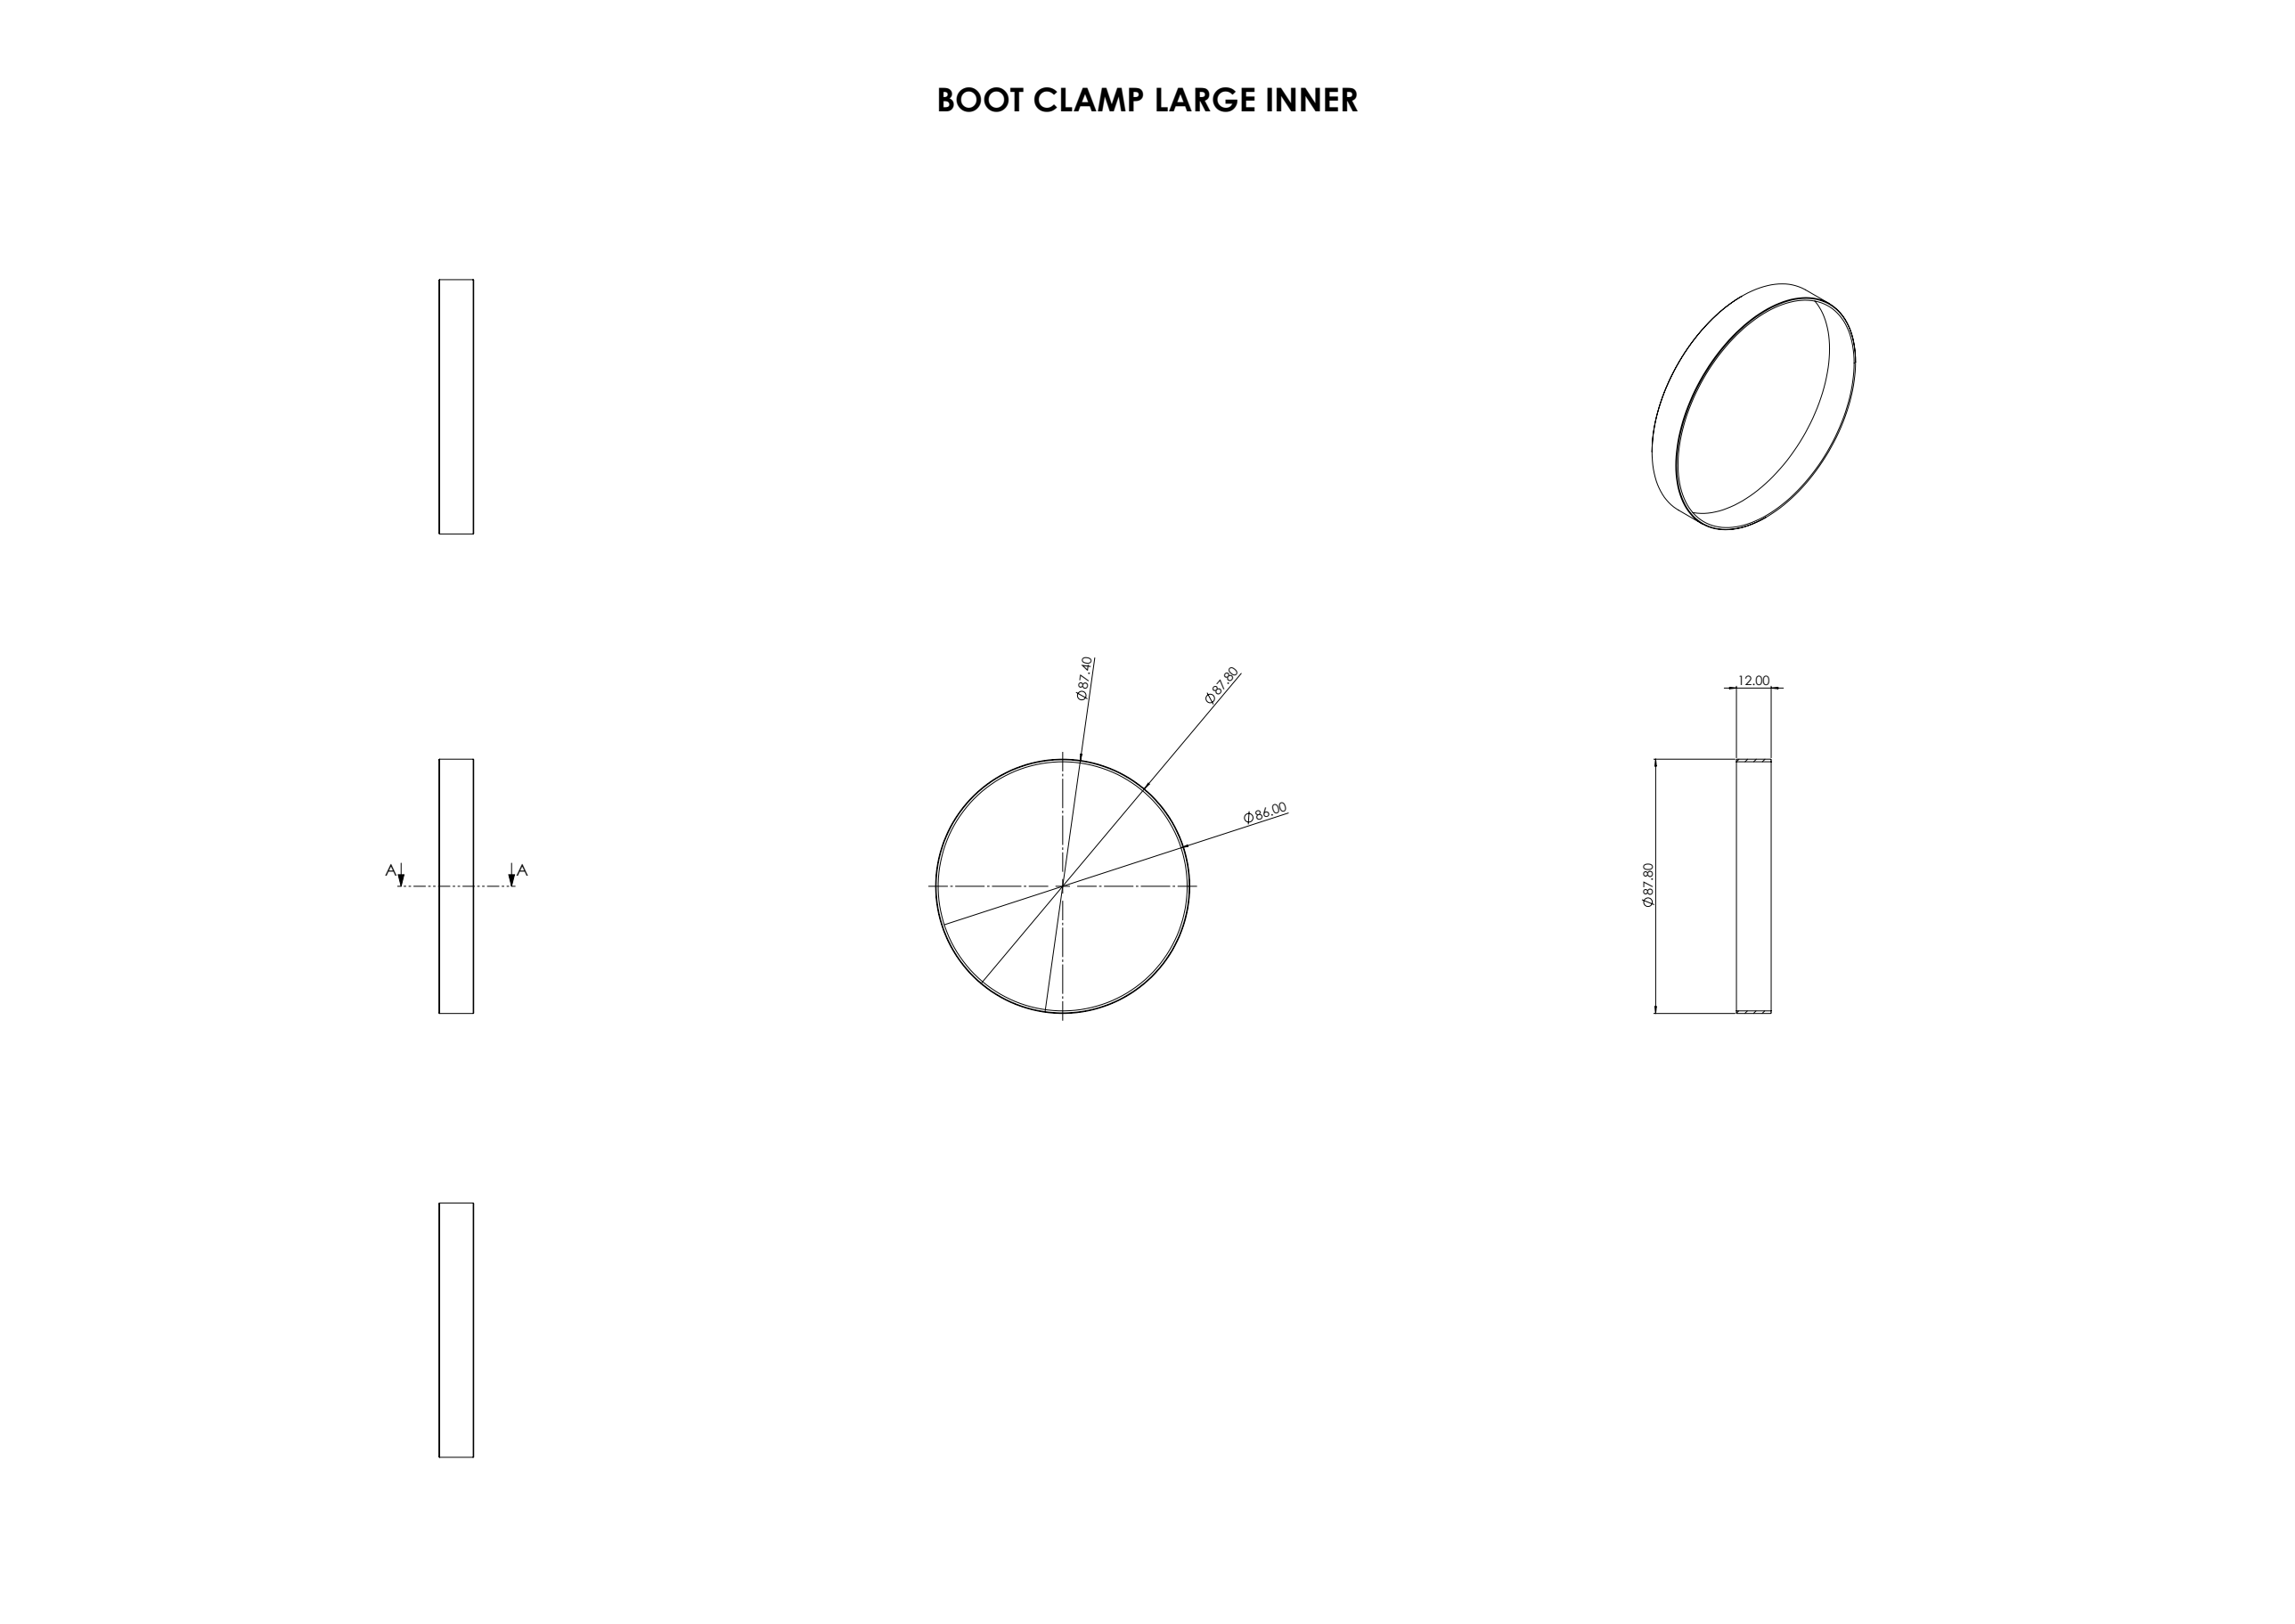
ISO-10303-21;
HEADER;
/* Generated by software containing ST-Developer
 * from STEP Tools, Inc. (www.steptools.com) 
 */

FILE_DESCRIPTION(
/* description */ (''),
/* implementation_level */ '2;1');

FILE_NAME(
/* name */ '12_Boot_Clamp_Large_Inner.step',
/* time_stamp */ '2026-10-11T12:57:03-07:00',
/* author */ (''),
/* organization */ (''),
/* preprocessor_version */ 'ST-DEVELOPER v20.2',
/* originating_system */ 'Autodesk Translation Framework v15.15.0.0',
/* authorisation */ '');

FILE_SCHEMA (('AUTOMOTIVE_DESIGN { 1 0 10303 214 3 1 1 }'));
ENDSEC;

DATA;
#10=MECHANICAL_DESIGN_GEOMETRIC_PRESENTATION_REPRESENTATION('',(#267),#90374);
#233=SHAPE_REPRESENTATION_RELATIONSHIP('SRR','None',#90452,#250);
#250=ADVANCED_BREP_SHAPE_REPRESENTATION('',(#284),#90368);
#267=STYLED_ITEM('',(#90673),#284);
#284=MANIFOLD_SOLID_BREP('Body1',#40356);
#743=CONICAL_SURFACE('',#44259,43.8,0.785398163397559);
#744=CONICAL_SURFACE('',#44264,43.8,0.785398163397382);
#1075=FACE_BOUND('',#6518,.T.);
#1076=FACE_BOUND('',#6521,.T.);
#1639=PLANE('',#44266);
#1640=PLANE('',#44270);
#4082=FACE_OUTER_BOUND('',#6514,.T.);
#4083=FACE_OUTER_BOUND('',#6515,.T.);
#4084=FACE_OUTER_BOUND('',#6516,.T.);
#4085=FACE_OUTER_BOUND('',#6517,.T.);
#4086=FACE_OUTER_BOUND('',#6519,.T.);
#4087=FACE_OUTER_BOUND('',#6520,.T.);
#6514=EDGE_LOOP('',(#34841,#34842,#34843,#34844));
#6515=EDGE_LOOP('',(#34845,#34846,#34847,#34848));
#6516=EDGE_LOOP('',(#34849,#34850,#34851,#34852));
#6517=EDGE_LOOP('',(#34853));
#6518=EDGE_LOOP('',(#34854));
#6519=EDGE_LOOP('',(#34855,#34856,#34857,#34858));
#6520=EDGE_LOOP('',(#34859));
#6521=EDGE_LOOP('',(#34860));
#8865=CIRCLE('',#44260,43.9);
#8866=CIRCLE('',#44261,43.7);
#8867=CIRCLE('',#44263,43.9);
#8868=CIRCLE('',#44265,43.7);
#8869=CIRCLE('',#44267,43.);
#8870=CIRCLE('',#44269,43.);
#12342=LINE('',#86910,#14836);
#12343=LINE('',#86915,#14837);
#12344=LINE('',#86919,#14838);
#12345=LINE('',#86925,#14839);
#14836=VECTOR('',#54702,43.8);
#14837=VECTOR('',#54709,43.9);
#14838=VECTOR('',#54714,43.8);
#14839=VECTOR('',#54721,43.);
#18296=VERTEX_POINT('',#86907);
#18297=VERTEX_POINT('',#86909);
#18298=VERTEX_POINT('',#86913);
#18299=VERTEX_POINT('',#86917);
#18300=VERTEX_POINT('',#86921);
#18301=VERTEX_POINT('',#86924);
#23932=EDGE_CURVE('',#18296,#18296,#8865,.T.);
#23933=EDGE_CURVE('',#18296,#18297,#12342,.T.);
#23934=EDGE_CURVE('',#18297,#18297,#8866,.T.);
#23935=EDGE_CURVE('',#18298,#18298,#8867,.T.);
#23936=EDGE_CURVE('',#18298,#18296,#12343,.T.);
#23937=EDGE_CURVE('',#18299,#18299,#8868,.T.);
#23938=EDGE_CURVE('',#18299,#18298,#12344,.T.);
#23939=EDGE_CURVE('',#18300,#18300,#8869,.T.);
#23940=EDGE_CURVE('',#18300,#18301,#12345,.T.);
#23941=EDGE_CURVE('',#18301,#18301,#8870,.T.);
#34841=ORIENTED_EDGE('',*,*,#23932,.F.);
#34842=ORIENTED_EDGE('',*,*,#23933,.T.);
#34843=ORIENTED_EDGE('',*,*,#23934,.T.);
#34844=ORIENTED_EDGE('',*,*,#23933,.F.);
#34845=ORIENTED_EDGE('',*,*,#23935,.F.);
#34846=ORIENTED_EDGE('',*,*,#23936,.T.);
#34847=ORIENTED_EDGE('',*,*,#23932,.T.);
#34848=ORIENTED_EDGE('',*,*,#23936,.F.);
#34849=ORIENTED_EDGE('',*,*,#23937,.F.);
#34850=ORIENTED_EDGE('',*,*,#23938,.T.);
#34851=ORIENTED_EDGE('',*,*,#23935,.T.);
#34852=ORIENTED_EDGE('',*,*,#23938,.F.);
#34853=ORIENTED_EDGE('',*,*,#23937,.T.);
#34854=ORIENTED_EDGE('',*,*,#23939,.F.);
#34855=ORIENTED_EDGE('',*,*,#23939,.T.);
#34856=ORIENTED_EDGE('',*,*,#23940,.T.);
#34857=ORIENTED_EDGE('',*,*,#23941,.F.);
#34858=ORIENTED_EDGE('',*,*,#23940,.F.);
#34859=ORIENTED_EDGE('',*,*,#23934,.F.);
#34860=ORIENTED_EDGE('',*,*,#23941,.T.);
#37783=CYLINDRICAL_SURFACE('',#44262,43.9);
#37784=CYLINDRICAL_SURFACE('',#44268,43.);
#39885=ADVANCED_FACE('',(#4082),#743,.T.);
#39886=ADVANCED_FACE('',(#4083),#37783,.T.);
#39887=ADVANCED_FACE('',(#4084),#744,.T.);
#39888=ADVANCED_FACE('',(#4085,#1075),#1639,.T.);
#39889=ADVANCED_FACE('',(#4086),#37784,.F.);
#39890=ADVANCED_FACE('',(#4087,#1076),#1640,.T.);
#40356=CLOSED_SHELL('',(#39885,#39886,#39887,#39888,#39889,#39890));
#44258=AXIS2_PLACEMENT_3D('',#86905,#54696,#54697);
#44259=AXIS2_PLACEMENT_3D('',#86906,#54698,#54699);
#44260=AXIS2_PLACEMENT_3D('',#86908,#54700,#54701);
#44261=AXIS2_PLACEMENT_3D('',#86911,#54703,#54704);
#44262=AXIS2_PLACEMENT_3D('',#86912,#54705,#54706);
#44263=AXIS2_PLACEMENT_3D('',#86914,#54707,#54708);
#44264=AXIS2_PLACEMENT_3D('',#86916,#54710,#54711);
#44265=AXIS2_PLACEMENT_3D('',#86918,#54712,#54713);
#44266=AXIS2_PLACEMENT_3D('',#86920,#54715,#54716);
#44267=AXIS2_PLACEMENT_3D('',#86922,#54717,#54718);
#44268=AXIS2_PLACEMENT_3D('',#86923,#54719,#54720);
#44269=AXIS2_PLACEMENT_3D('',#86926,#54722,#54723);
#44270=AXIS2_PLACEMENT_3D('',#86927,#54724,#54725);
#54696=DIRECTION('axis',(0.,0.,1.));
#54697=DIRECTION('refdir',(1.,0.,0.));
#54698=DIRECTION('center_axis',(1.,0.,0.));
#54699=DIRECTION('ref_axis',(0.,1.,0.));
#54700=DIRECTION('center_axis',(1.,0.,0.));
#54701=DIRECTION('ref_axis',(0.,0.,-1.));
#54702=DIRECTION('',(-0.707106781186469,0.707106781186626,8.65956056235589E-17));
#54703=DIRECTION('center_axis',(1.,0.,0.));
#54704=DIRECTION('ref_axis',(0.,0.,-1.));
#54705=DIRECTION('center_axis',(1.,0.,0.));
#54706=DIRECTION('ref_axis',(0.,1.,0.));
#54707=DIRECTION('center_axis',(1.,0.,0.));
#54708=DIRECTION('ref_axis',(0.,0.,-1.));
#54709=DIRECTION('',(-1.,0.,0.));
#54710=DIRECTION('center_axis',(-1.,0.,0.));
#54711=DIRECTION('ref_axis',(0.,1.,0.));
#54712=DIRECTION('center_axis',(1.,0.,0.));
#54713=DIRECTION('ref_axis',(0.,0.,-1.));
#54714=DIRECTION('',(-0.707106781186595,-0.7071067811865,-8.65956056235436E-17));
#54715=DIRECTION('center_axis',(1.,0.,0.));
#54716=DIRECTION('ref_axis',(0.,0.,-1.));
#54717=DIRECTION('center_axis',(1.,0.,0.));
#54718=DIRECTION('ref_axis',(0.,0.,-1.));
#54719=DIRECTION('center_axis',(1.,0.,0.));
#54720=DIRECTION('ref_axis',(0.,1.,0.));
#54721=DIRECTION('',(-1.,0.,0.));
#54722=DIRECTION('center_axis',(1.,0.,0.));
#54723=DIRECTION('ref_axis',(0.,0.,-1.));
#54724=DIRECTION('center_axis',(-1.,0.,0.));
#54725=DIRECTION('ref_axis',(0.,0.,1.));
#86905=CARTESIAN_POINT('',(0.,0.,0.));
#86906=CARTESIAN_POINT('Origin',(501.1,0.,0.));
#86907=CARTESIAN_POINT('',(501.2,-43.9,-5.37619944825688E-15));
#86908=CARTESIAN_POINT('Origin',(501.2,0.,0.));
#86909=CARTESIAN_POINT('',(501.,-43.7,-5.35170651227393E-15));
#86910=CARTESIAN_POINT('',(501.1,-43.8,-5.36395298026541E-15));
#86911=CARTESIAN_POINT('Origin',(501.,0.,0.));
#86912=CARTESIAN_POINT('Origin',(507.,0.,0.));
#86913=CARTESIAN_POINT('',(512.8,-43.9,-5.37619944825688E-15));
#86914=CARTESIAN_POINT('Origin',(512.8,0.,0.));
#86915=CARTESIAN_POINT('',(507.,-43.9,-5.37619944825688E-15));
#86916=CARTESIAN_POINT('Origin',(512.9,0.,0.));
#86917=CARTESIAN_POINT('',(513.,-43.7,-5.35170651227393E-15));
#86918=CARTESIAN_POINT('Origin',(513.,0.,0.));
#86919=CARTESIAN_POINT('',(512.9,-43.8,-5.36395298026541E-15));
#86920=CARTESIAN_POINT('Origin',(513.,43.,0.));
#86921=CARTESIAN_POINT('',(513.,-43.,-5.26598123633362E-15));
#86922=CARTESIAN_POINT('Origin',(513.,0.,0.));
#86923=CARTESIAN_POINT('Origin',(507.,0.,0.));
#86924=CARTESIAN_POINT('',(501.,-43.,-5.26598123633362E-15));
#86925=CARTESIAN_POINT('',(507.,-43.,-5.26598123633362E-15));
#86926=CARTESIAN_POINT('Origin',(501.,0.,0.));
#86927=CARTESIAN_POINT('Origin',(501.,43.7,0.));
#90349=UNCERTAINTY_MEASURE_WITH_UNIT(LENGTH_MEASURE(0.01),#90375,
'DISTANCE_ACCURACY_VALUE',
'Maximum model space distance between geometric entities at asserted c
onnectivities');
#90355=UNCERTAINTY_MEASURE_WITH_UNIT(LENGTH_MEASURE(0.01),#90375,
'DISTANCE_ACCURACY_VALUE',
'Maximum model space distance between geometric entities at asserted c
onnectivities');
#90368=(
GEOMETRIC_REPRESENTATION_CONTEXT(3)
GLOBAL_UNCERTAINTY_ASSIGNED_CONTEXT((#90349))
GLOBAL_UNIT_ASSIGNED_CONTEXT((#90375,#90377,#90378))
REPRESENTATION_CONTEXT('','3D')
);
#90374=(
GEOMETRIC_REPRESENTATION_CONTEXT(3)
GLOBAL_UNCERTAINTY_ASSIGNED_CONTEXT((#90355))
GLOBAL_UNIT_ASSIGNED_CONTEXT((#90375,#90377,#90378))
REPRESENTATION_CONTEXT('','3D')
);
#90375=(
LENGTH_UNIT()
NAMED_UNIT(*)
SI_UNIT(.MILLI.,.METRE.)
);
#90377=(
NAMED_UNIT(*)
PLANE_ANGLE_UNIT()
SI_UNIT($,.RADIAN.)
);
#90378=(
NAMED_UNIT(*)
SI_UNIT($,.STERADIAN.)
SOLID_ANGLE_UNIT()
);
#90391=SHAPE_DEFINITION_REPRESENTATION(#90409,#90452);
#90409=PRODUCT_DEFINITION_SHAPE('',$,#90471);
#90452=SHAPE_REPRESENTATION('',(#44258),#90368);
#90458=PRODUCT_DEFINITION_CONTEXT('part definition',#90514,'design');
#90471=PRODUCT_DEFINITION('2026-10-11-12-53-13-022',
'12_Boot_Clamp_Large_Inner',#90489,#90458);
#90489=PRODUCT_DEFINITION_FORMATION('',$,#90528);
#90514=APPLICATION_CONTEXT(
'Core Data for Automotive Mechanical Design Process');
#90515=PRODUCT_CONTEXT('part definition',#90514,'mechanical');
#90528=PRODUCT('2026-10-11-12-53-13-022','12_Boot_Clamp_Large_Inner',$,
(#90515));
#90667=COLOUR_RGB('Light Blue',0.38,0.62,0.78);
#90668=FILL_AREA_STYLE_COLOUR('',#90667);
#90669=FILL_AREA_STYLE('',(#90668));
#90670=SURFACE_STYLE_FILL_AREA(#90669);
#90671=SURFACE_SIDE_STYLE('',(#90670));
#90672=SURFACE_STYLE_USAGE(.BOTH.,#90671);
#90673=PRESENTATION_STYLE_ASSIGNMENT((#90672));
ENDSEC;
END-ISO-10303-21;
